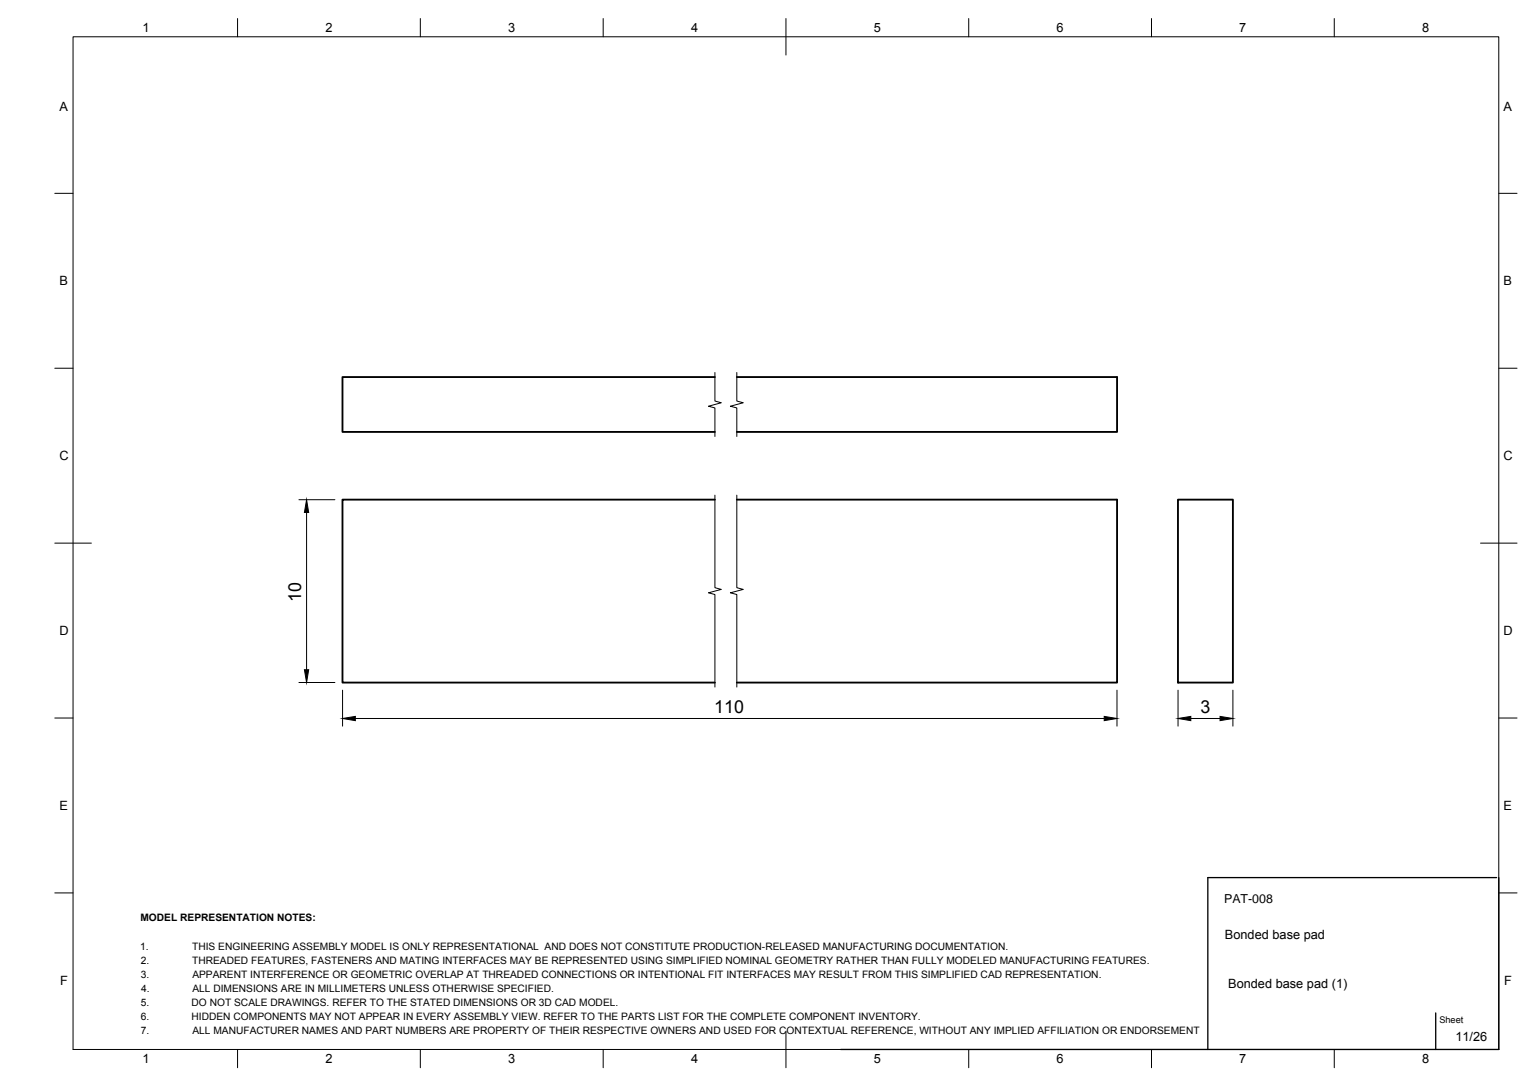
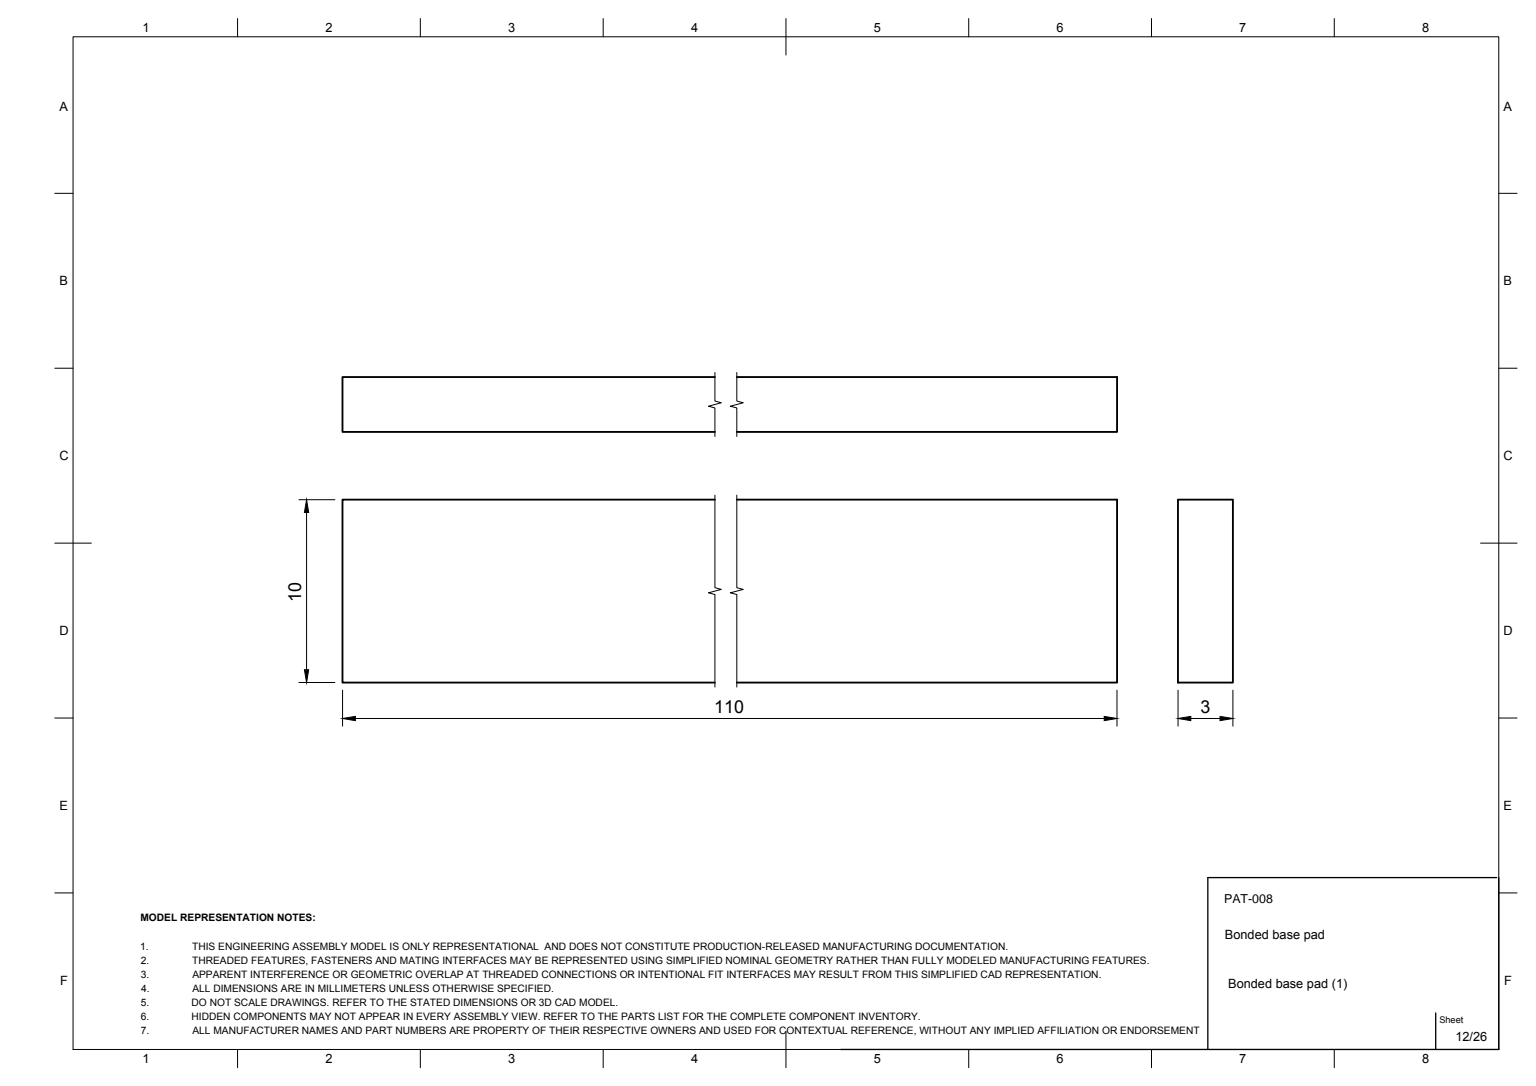
ISO-10303-21;
HEADER;
/* Generated by software containing ST-Developer
 * from STEP Tools, Inc. (www.steptools.com) 
 */

FILE_DESCRIPTION(
/* description */ ('Bearing housing with oil seal and end cap'),
/* implementation_level */ '2;1');

FILE_NAME(
/* name */ 'Bonded base pad.step',
/* time_stamp */ '2026-10-28T03:23:10-07:00',
/* author */ (''),
/* organization */ (''),
/* preprocessor_version */ 'ST-DEVELOPER v20.2',
/* originating_system */ 'Autodesk Translation Framework v15.17.0.0',
/* authorisation */ '');

FILE_SCHEMA (('AUTOMOTIVE_DESIGN { 1 0 10303 214 3 1 1 }'));
ENDSEC;

DATA;
#10=MECHANICAL_DESIGN_GEOMETRIC_PRESENTATION_REPRESENTATION('',(#265),#7871);
#223=SHAPE_REPRESENTATION_RELATIONSHIP('SRR','None',#7970,#244);
#244=ADVANCED_BREP_SHAPE_REPRESENTATION('',(#294),#7854);
#265=STYLED_ITEM('',(#8132),#294);
#294=MANIFOLD_SOLID_BREP('Body1',#4091);
#459=PLANE('',#4542);
#460=PLANE('',#4543);
#461=PLANE('',#4544);
#462=PLANE('',#4545);
#463=PLANE('',#4546);
#464=PLANE('',#4547);
#645=FACE_OUTER_BOUND('',#955,.T.);
#646=FACE_OUTER_BOUND('',#956,.T.);
#647=FACE_OUTER_BOUND('',#957,.T.);
#648=FACE_OUTER_BOUND('',#958,.T.);
#649=FACE_OUTER_BOUND('',#959,.T.);
#650=FACE_OUTER_BOUND('',#960,.T.);
#955=EDGE_LOOP('',(#3107,#3108,#3109,#3110));
#956=EDGE_LOOP('',(#3111,#3112,#3113,#3114));
#957=EDGE_LOOP('',(#3115,#3116,#3117,#3118));
#958=EDGE_LOOP('',(#3119,#3120,#3121,#3122));
#959=EDGE_LOOP('',(#3123,#3124,#3125,#3126));
#960=EDGE_LOOP('',(#3127,#3128,#3129,#3130));
#1237=LINE('',#6613,#1499);
#1238=LINE('',#6615,#1500);
#1239=LINE('',#6617,#1501);
#1240=LINE('',#6618,#1502);
#1241=LINE('',#6621,#1503);
#1242=LINE('',#6623,#1504);
#1243=LINE('',#6624,#1505);
#1244=LINE('',#6627,#1506);
#1245=LINE('',#6629,#1507);
#1246=LINE('',#6630,#1508);
#1247=LINE('',#6632,#1509);
#1248=LINE('',#6633,#1510);
#1499=VECTOR('',#5360,1.);
#1500=VECTOR('',#5361,1.);
#1501=VECTOR('',#5362,1.);
#1502=VECTOR('',#5363,1.);
#1503=VECTOR('',#5366,1.);
#1504=VECTOR('',#5367,1.);
#1505=VECTOR('',#5368,1.);
#1506=VECTOR('',#5371,1.);
#1507=VECTOR('',#5372,1.);
#1508=VECTOR('',#5373,1.);
#1509=VECTOR('',#5376,1.);
#1510=VECTOR('',#5377,1.);
#2011=VERTEX_POINT('',#6611);
#2012=VERTEX_POINT('',#6612);
#2013=VERTEX_POINT('',#6614);
#2014=VERTEX_POINT('',#6616);
#2015=VERTEX_POINT('',#6620);
#2016=VERTEX_POINT('',#6622);
#2017=VERTEX_POINT('',#6626);
#2018=VERTEX_POINT('',#6628);
#2417=EDGE_CURVE('',#2011,#2012,#1237,.T.);
#2418=EDGE_CURVE('',#2012,#2013,#1238,.T.);
#2419=EDGE_CURVE('',#2014,#2013,#1239,.T.);
#2420=EDGE_CURVE('',#2011,#2014,#1240,.T.);
#2421=EDGE_CURVE('',#2015,#2011,#1241,.T.);
#2422=EDGE_CURVE('',#2016,#2014,#1242,.T.);
#2423=EDGE_CURVE('',#2015,#2016,#1243,.T.);
#2424=EDGE_CURVE('',#2017,#2015,#1244,.T.);
#2425=EDGE_CURVE('',#2018,#2016,#1245,.T.);
#2426=EDGE_CURVE('',#2017,#2018,#1246,.T.);
#2427=EDGE_CURVE('',#2012,#2017,#1247,.T.);
#2428=EDGE_CURVE('',#2013,#2018,#1248,.T.);
#3107=ORIENTED_EDGE('',*,*,#2417,.T.);
#3108=ORIENTED_EDGE('',*,*,#2418,.T.);
#3109=ORIENTED_EDGE('',*,*,#2419,.F.);
#3110=ORIENTED_EDGE('',*,*,#2420,.F.);
#3111=ORIENTED_EDGE('',*,*,#2421,.T.);
#3112=ORIENTED_EDGE('',*,*,#2420,.T.);
#3113=ORIENTED_EDGE('',*,*,#2422,.F.);
#3114=ORIENTED_EDGE('',*,*,#2423,.F.);
#3115=ORIENTED_EDGE('',*,*,#2424,.T.);
#3116=ORIENTED_EDGE('',*,*,#2423,.T.);
#3117=ORIENTED_EDGE('',*,*,#2425,.F.);
#3118=ORIENTED_EDGE('',*,*,#2426,.F.);
#3119=ORIENTED_EDGE('',*,*,#2427,.T.);
#3120=ORIENTED_EDGE('',*,*,#2426,.T.);
#3121=ORIENTED_EDGE('',*,*,#2428,.F.);
#3122=ORIENTED_EDGE('',*,*,#2418,.F.);
#3123=ORIENTED_EDGE('',*,*,#2428,.T.);
#3124=ORIENTED_EDGE('',*,*,#2425,.T.);
#3125=ORIENTED_EDGE('',*,*,#2422,.T.);
#3126=ORIENTED_EDGE('',*,*,#2419,.T.);
#3127=ORIENTED_EDGE('',*,*,#2427,.F.);
#3128=ORIENTED_EDGE('',*,*,#2417,.F.);
#3129=ORIENTED_EDGE('',*,*,#2421,.F.);
#3130=ORIENTED_EDGE('',*,*,#2424,.F.);
#3927=ADVANCED_FACE('',(#645),#459,.T.);
#3928=ADVANCED_FACE('',(#646),#460,.T.);
#3929=ADVANCED_FACE('',(#647),#461,.T.);
#3930=ADVANCED_FACE('',(#648),#462,.T.);
#3931=ADVANCED_FACE('',(#649),#463,.T.);
#3932=ADVANCED_FACE('',(#650),#464,.F.);
#4091=CLOSED_SHELL('',(#3927,#3928,#3929,#3930,#3931,#3932));
#4541=AXIS2_PLACEMENT_3D('',#6609,#5356,#5357);
#4542=AXIS2_PLACEMENT_3D('',#6610,#5358,#5359);
#4543=AXIS2_PLACEMENT_3D('',#6619,#5364,#5365);
#4544=AXIS2_PLACEMENT_3D('',#6625,#5369,#5370);
#4545=AXIS2_PLACEMENT_3D('',#6631,#5374,#5375);
#4546=AXIS2_PLACEMENT_3D('',#6634,#5378,#5379);
#4547=AXIS2_PLACEMENT_3D('',#6635,#5380,#5381);
#5356=DIRECTION('axis',(0.,0.,1.));
#5357=DIRECTION('refdir',(1.,0.,0.));
#5358=DIRECTION('center_axis',(0.,1.,0.));
#5359=DIRECTION('ref_axis',(-1.,0.,0.));
#5360=DIRECTION('',(-1.,0.,0.));
#5361=DIRECTION('',(0.,0.,1.));
#5362=DIRECTION('',(-1.,0.,0.));
#5363=DIRECTION('',(0.,0.,1.));
#5364=DIRECTION('center_axis',(1.,0.,0.));
#5365=DIRECTION('ref_axis',(0.,1.,0.));
#5366=DIRECTION('',(0.,1.,0.));
#5367=DIRECTION('',(0.,1.,0.));
#5368=DIRECTION('',(0.,0.,1.));
#5369=DIRECTION('center_axis',(0.,-1.,0.));
#5370=DIRECTION('ref_axis',(1.,0.,0.));
#5371=DIRECTION('',(1.,0.,0.));
#5372=DIRECTION('',(1.,0.,0.));
#5373=DIRECTION('',(0.,0.,1.));
#5374=DIRECTION('center_axis',(-1.,0.,0.));
#5375=DIRECTION('ref_axis',(0.,-1.,0.));
#5376=DIRECTION('',(0.,-1.,0.));
#5377=DIRECTION('',(0.,-1.,0.));
#5378=DIRECTION('center_axis',(0.,0.,1.));
#5379=DIRECTION('ref_axis',(1.,0.,0.));
#5380=DIRECTION('center_axis',(0.,0.,1.));
#5381=DIRECTION('ref_axis',(1.,0.,0.));
#6609=CARTESIAN_POINT('',(0.,0.,0.));
#6610=CARTESIAN_POINT('Origin',(5.5,0.,-0.3));
#6611=CARTESIAN_POINT('',(5.5,0.,-0.3));
#6612=CARTESIAN_POINT('',(-5.5,0.,-0.3));
#6613=CARTESIAN_POINT('',(5.5,0.,-0.3));
#6614=CARTESIAN_POINT('',(-5.5,0.,0.));
#6615=CARTESIAN_POINT('',(-5.5,0.,-0.3));
#6616=CARTESIAN_POINT('',(5.5,0.,0.));
#6617=CARTESIAN_POINT('',(5.5,0.,0.));
#6618=CARTESIAN_POINT('',(5.5,0.,-0.3));
#6619=CARTESIAN_POINT('Origin',(5.5,-1.,-0.3));
#6620=CARTESIAN_POINT('',(5.5,-1.,-0.3));
#6621=CARTESIAN_POINT('',(5.5,-1.,-0.3));
#6622=CARTESIAN_POINT('',(5.5,-1.,0.));
#6623=CARTESIAN_POINT('',(5.5,-1.,0.));
#6624=CARTESIAN_POINT('',(5.5,-1.,-0.3));
#6625=CARTESIAN_POINT('Origin',(-5.5,-1.,-0.3));
#6626=CARTESIAN_POINT('',(-5.5,-1.,-0.3));
#6627=CARTESIAN_POINT('',(-5.5,-1.,-0.3));
#6628=CARTESIAN_POINT('',(-5.5,-1.,0.));
#6629=CARTESIAN_POINT('',(-5.5,-1.,0.));
#6630=CARTESIAN_POINT('',(-5.5,-1.,-0.3));
#6631=CARTESIAN_POINT('Origin',(-5.5,0.,-0.3));
#6632=CARTESIAN_POINT('',(-5.5,0.,-0.3));
#6633=CARTESIAN_POINT('',(-5.5,0.,0.));
#6634=CARTESIAN_POINT('Origin',(0.,-0.5,0.));
#6635=CARTESIAN_POINT('Origin',(0.,-0.5,-0.3));
#7828=UNCERTAINTY_MEASURE_WITH_UNIT(LENGTH_MEASURE(0.001),#7872,
'DISTANCE_ACCURACY_VALUE',
'Maximum model space distance between geometric entities at asserted c
onnectivities');
#7845=UNCERTAINTY_MEASURE_WITH_UNIT(LENGTH_MEASURE(0.001),#7872,
'DISTANCE_ACCURACY_VALUE',
'Maximum model space distance between geometric entities at asserted c
onnectivities');
#7854=(
GEOMETRIC_REPRESENTATION_CONTEXT(3)
GLOBAL_UNCERTAINTY_ASSIGNED_CONTEXT((#7828))
GLOBAL_UNIT_ASSIGNED_CONTEXT((#7872,#7874,#7875))
REPRESENTATION_CONTEXT('','3D')
);
#7871=(
GEOMETRIC_REPRESENTATION_CONTEXT(3)
GLOBAL_UNCERTAINTY_ASSIGNED_CONTEXT((#7845))
GLOBAL_UNIT_ASSIGNED_CONTEXT((#7872,#7874,#7875))
REPRESENTATION_CONTEXT('','3D')
);
#7872=(
LENGTH_UNIT()
NAMED_UNIT(*)
SI_UNIT(.CENTI.,.METRE.)
);
#7874=(
NAMED_UNIT(*)
PLANE_ANGLE_UNIT()
SI_UNIT($,.RADIAN.)
);
#7875=(
NAMED_UNIT(*)
SI_UNIT($,.STERADIAN.)
SOLID_ANGLE_UNIT()
);
#7884=SHAPE_DEFINITION_REPRESENTATION(#7909,#7970);
#7909=PRODUCT_DEFINITION_SHAPE('',$,#7996);
#7970=SHAPE_REPRESENTATION('',(#4541),#7854);
#7987=PRODUCT_DEFINITION_CONTEXT('part definition',#8064,'design');
#7996=PRODUCT_DEFINITION('Bonded base pad','Bonded base pad',#8021,#7987);
#8021=PRODUCT_DEFINITION_FORMATION('',$,#8074);
#8064=APPLICATION_CONTEXT(
'Core Data for Automotive Mechanical Design Process');
#8065=PRODUCT_CONTEXT('part definition',#8064,'mechanical');
#8074=PRODUCT('Bonded base pad','Bonded base pad','Bonded base pad',(#8065));
#8126=COLOUR_RGB('Dark Blue',0.08,0.2,0.34);
#8127=FILL_AREA_STYLE_COLOUR('',#8126);
#8128=FILL_AREA_STYLE('',(#8127));
#8129=SURFACE_STYLE_FILL_AREA(#8128);
#8130=SURFACE_SIDE_STYLE('',(#8129));
#8131=SURFACE_STYLE_USAGE(.BOTH.,#8130);
#8132=PRESENTATION_STYLE_ASSIGNMENT((#8131));
ENDSEC;
END-ISO-10303-21;
